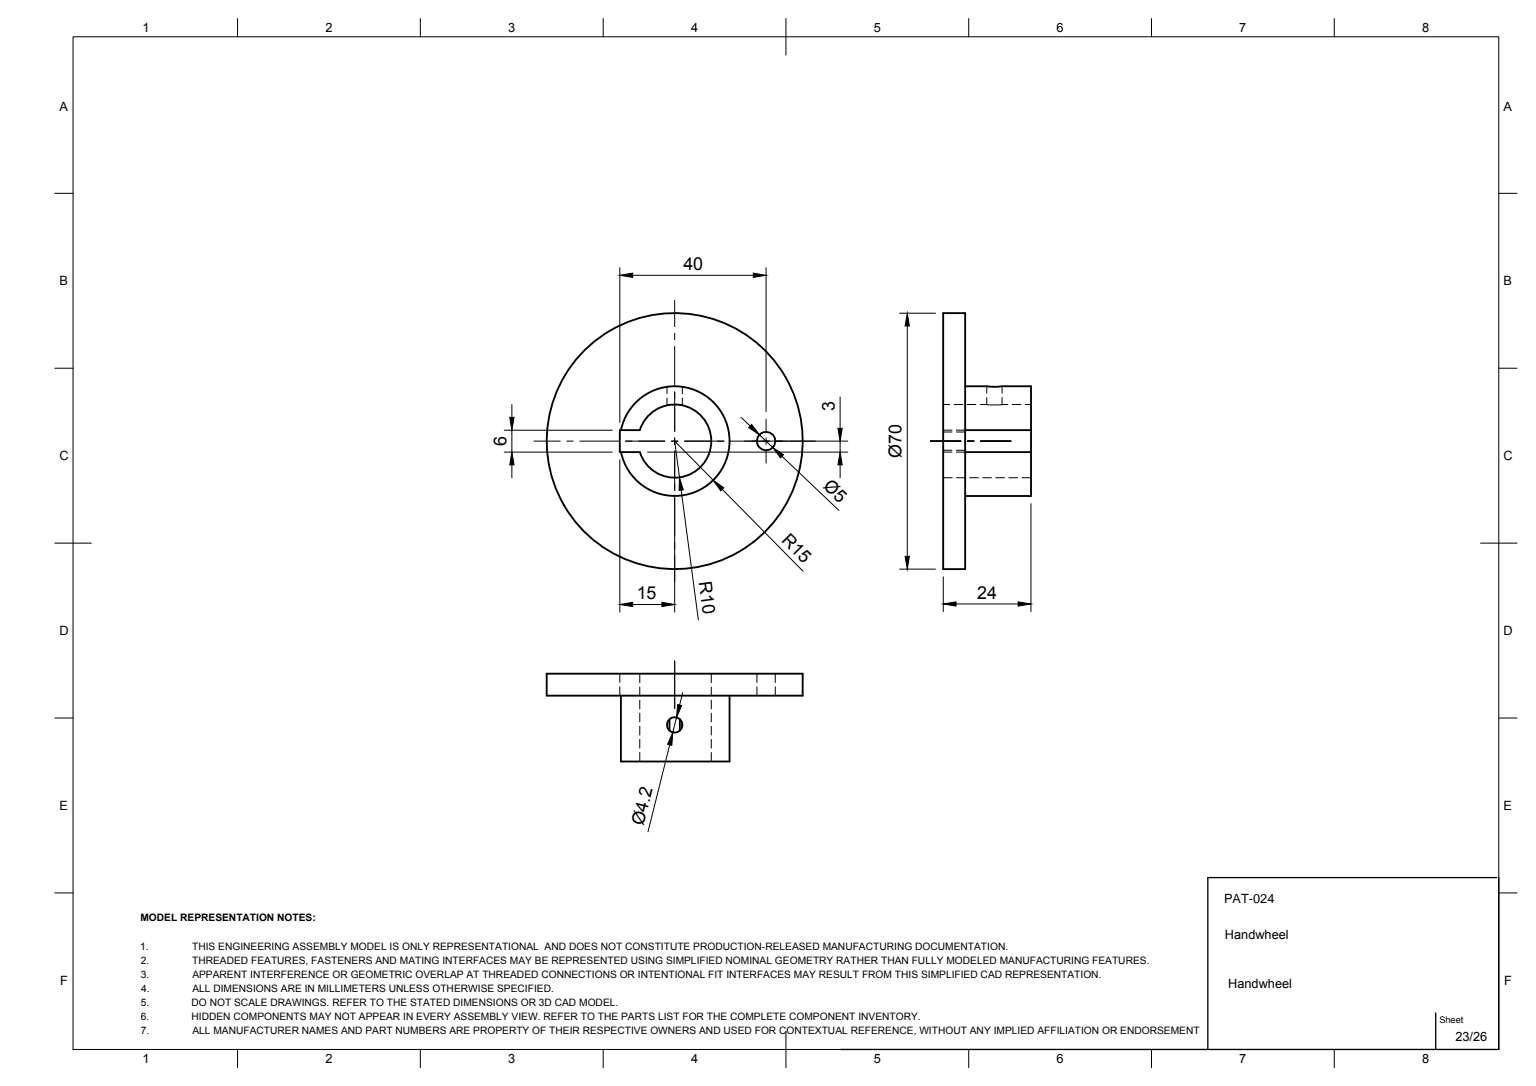
ISO-10303-21;
HEADER;
/* Generated by software containing ST-Developer
 * from STEP Tools, Inc. (www.steptools.com) 
 */

FILE_DESCRIPTION(
/* description */ ('Compact handwheel screw vise'),
/* implementation_level */ '2;1');

FILE_NAME(
/* name */ 'Handwheel.step',
/* time_stamp */ '2026-10-29T16:08:22-07:00',
/* author */ (''),
/* organization */ (''),
/* preprocessor_version */ 'ST-DEVELOPER v20.2',
/* originating_system */ 'Autodesk Translation Framework v15.17.0.0',
/* authorisation */ '');

FILE_SCHEMA (('AUTOMOTIVE_DESIGN { 1 0 10303 214 3 1 1 }'));
ENDSEC;

DATA;
#10=MECHANICAL_DESIGN_GEOMETRIC_PRESENTATION_REPRESENTATION('',(#673),#25074);
#536=B_SPLINE_CURVE_WITH_KNOTS('',3,(#24645,#24646,#24647,#24648,#24649,
#24650),.UNSPECIFIED.,.F.,.F.,(4,2,4),(0.803821788694078,0.872950991853625,
0.952307212900975),.UNSPECIFIED.);
#537=B_SPLINE_CURVE_WITH_KNOTS('',3,(#24653,#24654,#24655,#24656,#24657,
#24658,#24659,#24660,#24661,#24662),.UNSPECIFIED.,.F.,.F.,(4,2,2,2,4),(0.168950313426762,
0.238079516586309,0.317435737633658,0.396791958681008,0.465921161840561),
 .UNSPECIFIED.);
#538=B_SPLINE_CURVE_WITH_KNOTS('',3,(#24663,#24664,#24665,#24666,#24667,
#24668),.UNSPECIFIED.,.F.,.F.,(4,2,4),(0.952307212900975,1.03166343394832,
1.10079263710787),.UNSPECIFIED.);
#539=B_SPLINE_CURVE_WITH_KNOTS('',3,(#24672,#24673,#24674,#24675,#24676,
#24677,#24678,#24679,#24680,#24681),.UNSPECIFIED.,.F.,.F.,(4,2,2,2,4),(0.,
0.0792165807733642,0.158433161546728,0.237648697074572,0.316864232602417),
 .UNSPECIFIED.);
#540=B_SPLINE_CURVE_WITH_KNOTS('',3,(#24682,#24683,#24684,#24685,#24686,
#24687,#24688,#24689,#24690,#24691,#24692,#24693,#24694,#24695,#24696,#24697,
#24698,#24699,#24700,#24701,#24702,#24703,#24704,#24705,#24706,#24707),
 .UNSPECIFIED.,.F.,.F.,(4,2,2,2,2,2,2,2,2,2,2,2,4),(0.316864232602417,0.396079768130261,
0.475295303658105,0.554511884431469,0.633728465204833,0.712945045978197,
0.792161626751562,0.871377162279406,0.95059269780725,1.02980823333509,1.10902376886294,
1.1882403496363,1.26745693040967),.UNSPECIFIED.);
#609=SHAPE_REPRESENTATION_RELATIONSHIP('SRR','None',#25220,#637);
#637=ADVANCED_BREP_SHAPE_REPRESENTATION('',(#706),#25067);
#673=STYLED_ITEM('',(#25432),#706);
#706=MANIFOLD_SOLID_BREP('Body1',#8084);
#808=FACE_BOUND('',#1992,.T.);
#809=FACE_BOUND('',#1993,.T.);
#810=FACE_BOUND('',#1995,.T.);
#811=FACE_BOUND('',#1996,.T.);
#812=FACE_BOUND('',#1999,.T.);
#813=FACE_BOUND('',#2001,.T.);
#968=PLANE('',#9070);
#969=PLANE('',#9074);
#970=PLANE('',#9075);
#971=PLANE('',#9076);
#972=PLANE('',#9077);
#973=PLANE('',#9078);
#974=PLANE('',#9081);
#975=PLANE('',#9089);
#1418=FACE_OUTER_BOUND('',#1984,.T.);
#1419=FACE_OUTER_BOUND('',#1985,.T.);
#1420=FACE_OUTER_BOUND('',#1986,.T.);
#1421=FACE_OUTER_BOUND('',#1987,.T.);
#1422=FACE_OUTER_BOUND('',#1988,.T.);
#1423=FACE_OUTER_BOUND('',#1989,.T.);
#1424=FACE_OUTER_BOUND('',#1990,.T.);
#1425=FACE_OUTER_BOUND('',#1991,.T.);
#1426=FACE_OUTER_BOUND('',#1994,.T.);
#1427=FACE_OUTER_BOUND('',#1997,.T.);
#1428=FACE_OUTER_BOUND('',#1998,.T.);
#1429=FACE_OUTER_BOUND('',#2000,.T.);
#1430=FACE_OUTER_BOUND('',#2002,.T.);
#1984=EDGE_LOOP('',(#7079,#7080,#7081,#7082));
#1985=EDGE_LOOP('',(#7083,#7084));
#1986=EDGE_LOOP('',(#7085,#7086,#7087,#7088,#7089,#7090,#7091,#7092,#7093));
#1987=EDGE_LOOP('',(#7094,#7095));
#1988=EDGE_LOOP('',(#7096,#7097,#7098,#7099,#7100,#7101));
#1989=EDGE_LOOP('',(#7102,#7103,#7104,#7105));
#1990=EDGE_LOOP('',(#7106,#7107,#7108,#7109,#7110,#7111));
#1991=EDGE_LOOP('',(#7112));
#1992=EDGE_LOOP('',(#7113));
#1993=EDGE_LOOP('',(#7114,#7115,#7116,#7117));
#1994=EDGE_LOOP('',(#7118));
#1995=EDGE_LOOP('',(#7119));
#1996=EDGE_LOOP('',(#7120,#7121,#7122,#7123));
#1997=EDGE_LOOP('',(#7124,#7125,#7126,#7127));
#1998=EDGE_LOOP('',(#7128,#7129,#7130,#7131));
#1999=EDGE_LOOP('',(#7132,#7133,#7134,#7135,#7136));
#2000=EDGE_LOOP('',(#7137,#7138,#7139,#7140));
#2001=EDGE_LOOP('',(#7141,#7142));
#2002=EDGE_LOOP('',(#7143,#7144,#7145,#7146));
#2476=LINE('',#24635,#2984);
#2477=LINE('',#24640,#2985);
#2478=LINE('',#24670,#2986);
#2479=LINE('',#24709,#2987);
#2480=LINE('',#24713,#2988);
#2481=LINE('',#24715,#2989);
#2482=LINE('',#24717,#2990);
#2483=LINE('',#24719,#2991);
#2484=LINE('',#24721,#2992);
#2485=LINE('',#24722,#2993);
#2486=LINE('',#24725,#2994);
#2487=LINE('',#24727,#2995);
#2488=LINE('',#24728,#2996);
#2489=LINE('',#24731,#2997);
#2490=LINE('',#24733,#2998);
#2491=LINE('',#24735,#2999);
#2492=LINE('',#24737,#3000);
#2493=LINE('',#24738,#3001);
#2494=LINE('',#24748,#3002);
#2984=VECTOR('',#10954,0.25);
#2985=VECTOR('',#10959,1.);
#2986=VECTOR('',#10966,0.210000000000001);
#2987=VECTOR('',#10969,1.);
#2988=VECTOR('',#10972,1.);
#2989=VECTOR('',#10973,1.);
#2990=VECTOR('',#10974,1.);
#2991=VECTOR('',#10975,1.);
#2992=VECTOR('',#10976,1.);
#2993=VECTOR('',#10977,1.);
#2994=VECTOR('',#10980,1.);
#2995=VECTOR('',#10981,1.);
#2996=VECTOR('',#10982,1.);
#2997=VECTOR('',#10985,1.);
#2998=VECTOR('',#10986,1.);
#2999=VECTOR('',#10987,1.);
#3000=VECTOR('',#10988,1.);
#3001=VECTOR('',#10989,1.);
#3002=VECTOR('',#11004,3.5);
#3299=CIRCLE('',#9068,0.25);
#3300=CIRCLE('',#9069,0.25);
#3301=CIRCLE('',#9071,0.210000000000001);
#3302=CIRCLE('',#9073,0.210000000000001);
#3303=CIRCLE('',#9079,3.5);
#3304=CIRCLE('',#9080,1.);
#3305=CIRCLE('',#9082,3.5);
#3306=CIRCLE('',#9083,1.5);
#3307=CIRCLE('',#9086,1.);
#3308=CIRCLE('',#9088,1.5);
#3979=VERTEX_POINT('',#24632);
#3980=VERTEX_POINT('',#24634);
#3981=VERTEX_POINT('',#24638);
#3982=VERTEX_POINT('',#24639);
#3983=VERTEX_POINT('',#24643);
#3984=VERTEX_POINT('',#24644);
#3985=VERTEX_POINT('',#24651);
#3986=VERTEX_POINT('',#24669);
#3987=VERTEX_POINT('',#24671);
#3988=VERTEX_POINT('',#24711);
#3989=VERTEX_POINT('',#24712);
#3990=VERTEX_POINT('',#24714);
#3991=VERTEX_POINT('',#24716);
#3992=VERTEX_POINT('',#24718);
#3993=VERTEX_POINT('',#24720);
#3994=VERTEX_POINT('',#24724);
#3995=VERTEX_POINT('',#24726);
#3996=VERTEX_POINT('',#24730);
#3997=VERTEX_POINT('',#24732);
#3998=VERTEX_POINT('',#24734);
#3999=VERTEX_POINT('',#24736);
#4000=VERTEX_POINT('',#24740);
#4001=VERTEX_POINT('',#24744);
#5026=EDGE_CURVE('',#3979,#3979,#3299,.T.);
#5027=EDGE_CURVE('',#3979,#3980,#2476,.T.);
#5028=EDGE_CURVE('',#3980,#3980,#3300,.T.);
#5029=EDGE_CURVE('',#3981,#3982,#2477,.T.);
#5030=EDGE_CURVE('',#3981,#3982,#3301,.T.);
#5031=EDGE_CURVE('',#3983,#3984,#536,.T.);
#5032=EDGE_CURVE('',#3985,#3983,#3302,.T.);
#5033=EDGE_CURVE('',#3982,#3985,#537,.T.);
#5034=EDGE_CURVE('',#3984,#3981,#538,.T.);
#5035=EDGE_CURVE('',#3984,#3986,#2478,.T.);
#5036=EDGE_CURVE('',#3987,#3986,#539,.T.);
#5037=EDGE_CURVE('',#3986,#3987,#540,.T.);
#5038=EDGE_CURVE('',#3985,#3983,#2479,.T.);
#5039=EDGE_CURVE('',#3988,#3989,#2480,.T.);
#5040=EDGE_CURVE('',#3990,#3988,#2481,.T.);
#5041=EDGE_CURVE('',#3991,#3990,#2482,.T.);
#5042=EDGE_CURVE('',#3992,#3991,#2483,.T.);
#5043=EDGE_CURVE('',#3993,#3992,#2484,.T.);
#5044=EDGE_CURVE('',#3989,#3993,#2485,.T.);
#5045=EDGE_CURVE('',#3994,#3988,#2486,.T.);
#5046=EDGE_CURVE('',#3995,#3994,#2487,.T.);
#5047=EDGE_CURVE('',#3990,#3995,#2488,.T.);
#5048=EDGE_CURVE('',#3996,#3994,#2489,.T.);
#5049=EDGE_CURVE('',#3997,#3996,#2490,.T.);
#5050=EDGE_CURVE('',#3998,#3997,#2491,.T.);
#5051=EDGE_CURVE('',#3999,#3998,#2492,.T.);
#5052=EDGE_CURVE('',#3995,#3999,#2493,.T.);
#5053=EDGE_CURVE('',#4000,#4000,#3303,.T.);
#5054=EDGE_CURVE('',#3989,#3996,#3304,.T.);
#5055=EDGE_CURVE('',#4001,#4001,#3305,.T.);
#5056=EDGE_CURVE('',#3999,#3991,#3306,.T.);
#5057=EDGE_CURVE('',#4000,#4001,#2494,.T.);
#5058=EDGE_CURVE('',#3993,#3997,#3307,.T.);
#5059=EDGE_CURVE('',#3998,#3992,#3308,.T.);
#7079=ORIENTED_EDGE('',*,*,#5026,.F.);
#7080=ORIENTED_EDGE('',*,*,#5027,.T.);
#7081=ORIENTED_EDGE('',*,*,#5028,.F.);
#7082=ORIENTED_EDGE('',*,*,#5027,.F.);
#7083=ORIENTED_EDGE('',*,*,#5029,.F.);
#7084=ORIENTED_EDGE('',*,*,#5030,.T.);
#7085=ORIENTED_EDGE('',*,*,#5031,.F.);
#7086=ORIENTED_EDGE('',*,*,#5032,.F.);
#7087=ORIENTED_EDGE('',*,*,#5033,.F.);
#7088=ORIENTED_EDGE('',*,*,#5030,.F.);
#7089=ORIENTED_EDGE('',*,*,#5034,.F.);
#7090=ORIENTED_EDGE('',*,*,#5035,.T.);
#7091=ORIENTED_EDGE('',*,*,#5036,.F.);
#7092=ORIENTED_EDGE('',*,*,#5037,.F.);
#7093=ORIENTED_EDGE('',*,*,#5035,.F.);
#7094=ORIENTED_EDGE('',*,*,#5038,.F.);
#7095=ORIENTED_EDGE('',*,*,#5032,.T.);
#7096=ORIENTED_EDGE('',*,*,#5039,.F.);
#7097=ORIENTED_EDGE('',*,*,#5040,.F.);
#7098=ORIENTED_EDGE('',*,*,#5041,.F.);
#7099=ORIENTED_EDGE('',*,*,#5042,.F.);
#7100=ORIENTED_EDGE('',*,*,#5043,.F.);
#7101=ORIENTED_EDGE('',*,*,#5044,.F.);
#7102=ORIENTED_EDGE('',*,*,#5045,.F.);
#7103=ORIENTED_EDGE('',*,*,#5046,.F.);
#7104=ORIENTED_EDGE('',*,*,#5047,.F.);
#7105=ORIENTED_EDGE('',*,*,#5040,.T.);
#7106=ORIENTED_EDGE('',*,*,#5048,.F.);
#7107=ORIENTED_EDGE('',*,*,#5049,.F.);
#7108=ORIENTED_EDGE('',*,*,#5050,.F.);
#7109=ORIENTED_EDGE('',*,*,#5051,.F.);
#7110=ORIENTED_EDGE('',*,*,#5052,.F.);
#7111=ORIENTED_EDGE('',*,*,#5046,.T.);
#7112=ORIENTED_EDGE('',*,*,#5053,.T.);
#7113=ORIENTED_EDGE('',*,*,#5028,.T.);
#7114=ORIENTED_EDGE('',*,*,#5048,.T.);
#7115=ORIENTED_EDGE('',*,*,#5045,.T.);
#7116=ORIENTED_EDGE('',*,*,#5039,.T.);
#7117=ORIENTED_EDGE('',*,*,#5054,.T.);
#7118=ORIENTED_EDGE('',*,*,#5055,.F.);
#7119=ORIENTED_EDGE('',*,*,#5026,.T.);
#7120=ORIENTED_EDGE('',*,*,#5052,.T.);
#7121=ORIENTED_EDGE('',*,*,#5056,.T.);
#7122=ORIENTED_EDGE('',*,*,#5041,.T.);
#7123=ORIENTED_EDGE('',*,*,#5047,.T.);
#7124=ORIENTED_EDGE('',*,*,#5053,.F.);
#7125=ORIENTED_EDGE('',*,*,#5057,.T.);
#7126=ORIENTED_EDGE('',*,*,#5055,.T.);
#7127=ORIENTED_EDGE('',*,*,#5057,.F.);
#7128=ORIENTED_EDGE('',*,*,#5049,.T.);
#7129=ORIENTED_EDGE('',*,*,#5054,.F.);
#7130=ORIENTED_EDGE('',*,*,#5044,.T.);
#7131=ORIENTED_EDGE('',*,*,#5058,.T.);
#7132=ORIENTED_EDGE('',*,*,#5033,.T.);
#7133=ORIENTED_EDGE('',*,*,#5038,.T.);
#7134=ORIENTED_EDGE('',*,*,#5031,.T.);
#7135=ORIENTED_EDGE('',*,*,#5034,.T.);
#7136=ORIENTED_EDGE('',*,*,#5029,.T.);
#7137=ORIENTED_EDGE('',*,*,#5051,.T.);
#7138=ORIENTED_EDGE('',*,*,#5059,.T.);
#7139=ORIENTED_EDGE('',*,*,#5042,.T.);
#7140=ORIENTED_EDGE('',*,*,#5056,.F.);
#7141=ORIENTED_EDGE('',*,*,#5036,.T.);
#7142=ORIENTED_EDGE('',*,*,#5037,.T.);
#7143=ORIENTED_EDGE('',*,*,#5050,.T.);
#7144=ORIENTED_EDGE('',*,*,#5058,.F.);
#7145=ORIENTED_EDGE('',*,*,#5043,.T.);
#7146=ORIENTED_EDGE('',*,*,#5059,.F.);
#7568=CYLINDRICAL_SURFACE('',#9067,0.25);
#7569=CYLINDRICAL_SURFACE('',#9072,0.210000000000001);
#7570=CYLINDRICAL_SURFACE('',#9084,3.5);
#7571=CYLINDRICAL_SURFACE('',#9085,1.);
#7572=CYLINDRICAL_SURFACE('',#9087,1.5);
#7988=ADVANCED_FACE('',(#1418),#7568,.F.);
#7989=ADVANCED_FACE('',(#1419),#968,.T.);
#7990=ADVANCED_FACE('',(#1420),#7569,.F.);
#7991=ADVANCED_FACE('',(#1421),#969,.T.);
#7992=ADVANCED_FACE('',(#1422),#970,.F.);
#7993=ADVANCED_FACE('',(#1423),#971,.F.);
#7994=ADVANCED_FACE('',(#1424),#972,.F.);
#7995=ADVANCED_FACE('',(#1425,#808,#809),#973,.T.);
#7996=ADVANCED_FACE('',(#1426,#810,#811),#974,.F.);
#7997=ADVANCED_FACE('',(#1427),#7570,.T.);
#7998=ADVANCED_FACE('',(#1428,#812),#7571,.F.);
#7999=ADVANCED_FACE('',(#1429,#813),#7572,.T.);
#8000=ADVANCED_FACE('',(#1430),#975,.F.);
#8084=CLOSED_SHELL('',(#7988,#7989,#7990,#7991,#7992,#7993,#7994,#7995,
#7996,#7997,#7998,#7999,#8000));
#9066=AXIS2_PLACEMENT_3D('',#24630,#10948,#10949);
#9067=AXIS2_PLACEMENT_3D('',#24631,#10950,#10951);
#9068=AXIS2_PLACEMENT_3D('',#24633,#10952,#10953);
#9069=AXIS2_PLACEMENT_3D('',#24636,#10955,#10956);
#9070=AXIS2_PLACEMENT_3D('',#24637,#10957,#10958);
#9071=AXIS2_PLACEMENT_3D('',#24641,#10960,#10961);
#9072=AXIS2_PLACEMENT_3D('',#24642,#10962,#10963);
#9073=AXIS2_PLACEMENT_3D('',#24652,#10964,#10965);
#9074=AXIS2_PLACEMENT_3D('',#24708,#10967,#10968);
#9075=AXIS2_PLACEMENT_3D('',#24710,#10970,#10971);
#9076=AXIS2_PLACEMENT_3D('',#24723,#10978,#10979);
#9077=AXIS2_PLACEMENT_3D('',#24729,#10983,#10984);
#9078=AXIS2_PLACEMENT_3D('',#24739,#10990,#10991);
#9079=AXIS2_PLACEMENT_3D('',#24741,#10992,#10993);
#9080=AXIS2_PLACEMENT_3D('',#24742,#10994,#10995);
#9081=AXIS2_PLACEMENT_3D('',#24743,#10996,#10997);
#9082=AXIS2_PLACEMENT_3D('',#24745,#10998,#10999);
#9083=AXIS2_PLACEMENT_3D('',#24746,#11000,#11001);
#9084=AXIS2_PLACEMENT_3D('',#24747,#11002,#11003);
#9085=AXIS2_PLACEMENT_3D('',#24749,#11005,#11006);
#9086=AXIS2_PLACEMENT_3D('',#24750,#11007,#11008);
#9087=AXIS2_PLACEMENT_3D('',#24751,#11009,#11010);
#9088=AXIS2_PLACEMENT_3D('',#24752,#11011,#11012);
#9089=AXIS2_PLACEMENT_3D('',#24753,#11013,#11014);
#10948=DIRECTION('axis',(0.,0.,1.));
#10949=DIRECTION('refdir',(1.,0.,0.));
#10950=DIRECTION('center_axis',(1.,0.,0.));
#10951=DIRECTION('ref_axis',(0.,0.,-1.));
#10952=DIRECTION('center_axis',(1.,0.,0.));
#10953=DIRECTION('ref_axis',(0.,0.,-1.));
#10954=DIRECTION('',(1.,0.,0.));
#10955=DIRECTION('center_axis',(-1.,0.,0.));
#10956=DIRECTION('ref_axis',(0.,0.,-1.));
#10957=DIRECTION('center_axis',(0.,1.,0.));
#10958=DIRECTION('ref_axis',(1.,0.,0.));
#10959=DIRECTION('',(1.,0.,0.));
#10960=DIRECTION('center_axis',(0.,1.,0.));
#10961=DIRECTION('ref_axis',(1.,0.,0.));
#10962=DIRECTION('center_axis',(0.,1.,0.));
#10963=DIRECTION('ref_axis',(1.,0.,0.));
#10964=DIRECTION('center_axis',(0.,1.,0.));
#10965=DIRECTION('ref_axis',(1.,0.,0.));
#10966=DIRECTION('',(0.,1.,0.));
#10967=DIRECTION('center_axis',(0.,1.,0.));
#10968=DIRECTION('ref_axis',(1.,0.,0.));
#10969=DIRECTION('',(-1.,0.,0.));
#10970=DIRECTION('center_axis',(0.,-1.,0.));
#10971=DIRECTION('ref_axis',(0.,0.,-1.));
#10972=DIRECTION('',(0.,0.,1.));
#10973=DIRECTION('',(1.,0.,0.));
#10974=DIRECTION('',(0.,0.,-1.));
#10975=DIRECTION('',(1.,0.,0.));
#10976=DIRECTION('',(0.,0.,-1.));
#10977=DIRECTION('',(-1.,0.,0.));
#10978=DIRECTION('center_axis',(0.,0.,-1.));
#10979=DIRECTION('ref_axis',(0.,1.,0.));
#10980=DIRECTION('',(0.,-1.,0.));
#10981=DIRECTION('',(1.,0.,0.));
#10982=DIRECTION('',(0.,1.,0.));
#10983=DIRECTION('center_axis',(0.,1.,0.));
#10984=DIRECTION('ref_axis',(0.,0.,1.));
#10985=DIRECTION('',(0.,0.,-1.));
#10986=DIRECTION('',(1.,0.,0.));
#10987=DIRECTION('',(0.,0.,1.));
#10988=DIRECTION('',(-1.,0.,0.));
#10989=DIRECTION('',(0.,0.,1.));
#10990=DIRECTION('center_axis',(1.,0.,0.));
#10991=DIRECTION('ref_axis',(0.,0.,-1.));
#10992=DIRECTION('center_axis',(1.,0.,0.));
#10993=DIRECTION('ref_axis',(0.,0.,-1.));
#10994=DIRECTION('center_axis',(-1.,0.,0.));
#10995=DIRECTION('ref_axis',(0.,0.,-1.));
#10996=DIRECTION('center_axis',(1.,0.,0.));
#10997=DIRECTION('ref_axis',(0.,0.,-1.));
#10998=DIRECTION('center_axis',(1.,0.,0.));
#10999=DIRECTION('ref_axis',(0.,0.,-1.));
#11000=DIRECTION('center_axis',(1.,0.,0.));
#11001=DIRECTION('ref_axis',(0.,0.,-1.));
#11002=DIRECTION('center_axis',(1.,0.,0.));
#11003=DIRECTION('ref_axis',(0.,0.,-1.));
#11004=DIRECTION('',(-1.,0.,0.));
#11005=DIRECTION('center_axis',(1.,0.,0.));
#11006=DIRECTION('ref_axis',(0.,1.22464679914735E-16,1.));
#11007=DIRECTION('center_axis',(-1.,0.,0.));
#11008=DIRECTION('ref_axis',(0.,0.,-1.));
#11009=DIRECTION('center_axis',(1.,0.,0.));
#11010=DIRECTION('ref_axis',(0.,1.22464679914735E-16,1.));
#11011=DIRECTION('center_axis',(1.,0.,0.));
#11012=DIRECTION('ref_axis',(0.,0.,-1.));
#11013=DIRECTION('center_axis',(1.,0.,0.));
#11014=DIRECTION('ref_axis',(0.,0.,-1.));
#24630=CARTESIAN_POINT('',(0.,0.,0.));
#24631=CARTESIAN_POINT('Origin',(28.7,0.,6.5));
#24632=CARTESIAN_POINT('',(28.8,-3.06161699786838E-17,6.75));
#24633=CARTESIAN_POINT('Origin',(28.8,0.,6.5));
#24634=CARTESIAN_POINT('',(29.4,3.06161699786838E-17,6.75));
#24635=CARTESIAN_POINT('',(28.7,-3.06161699786838E-17,6.75));
#24636=CARTESIAN_POINT('Origin',(29.4,0.,6.5));
#24637=CARTESIAN_POINT('Origin',(28.,0.99,4.));
#24638=CARTESIAN_POINT('',(27.844436508139,0.99,4.14106735979666));
#24639=CARTESIAN_POINT('',(28.155563491861,0.99,4.14106735979666));
#24640=CARTESIAN_POINT('',(27.,0.99,4.14106735979666));
#24641=CARTESIAN_POINT('Origin',(28.,0.99,4.));
#24642=CARTESIAN_POINT('Origin',(28.,0.99,4.));
#24643=CARTESIAN_POINT('',(27.844436508139,0.99,3.85893264020334));
#24644=CARTESIAN_POINT('',(27.79,1.,4.));
#24645=CARTESIAN_POINT('Ctrl Pts',(27.844436508139,0.99,3.85893264020334));
#24646=CARTESIAN_POINT('Ctrl Pts',(27.8287948476368,0.992457849824465,3.87618164330178));
#24647=CARTESIAN_POINT('Ctrl Pts',(27.815375956669,0.994938193049464,3.8970013568903));
#24648=CARTESIAN_POINT('Ctrl Pts',(27.7953025362756,0.998844492372413,3.94538588560165));
#24649=CARTESIAN_POINT('Ctrl Pts',(27.79,1.,3.97354792631755));
#24650=CARTESIAN_POINT('Ctrl Pts',(27.79,1.,4.));
#24651=CARTESIAN_POINT('',(28.155563491861,0.99,3.85893264020334));
#24652=CARTESIAN_POINT('Origin',(28.,0.99,4.));
#24653=CARTESIAN_POINT('Ctrl Pts',(28.155563491861,0.99,4.14106735979666));
#24654=CARTESIAN_POINT('Ctrl Pts',(28.1712051523632,0.992457849824465,4.12381835669823));
#24655=CARTESIAN_POINT('Ctrl Pts',(28.184624043331,0.994938193049464,4.1029986431097));
#24656=CARTESIAN_POINT('Ctrl Pts',(28.2046974637244,0.998844492372413,4.05461411439835));
#24657=CARTESIAN_POINT('Ctrl Pts',(28.21,1.,4.02645207368245));
#24658=CARTESIAN_POINT('Ctrl Pts',(28.21,1.,3.97354792631755));
#24659=CARTESIAN_POINT('Ctrl Pts',(28.2046974637244,0.998844492372413,3.94538588560165));
#24660=CARTESIAN_POINT('Ctrl Pts',(28.184624043331,0.994938193049464,3.8970013568903));
#24661=CARTESIAN_POINT('Ctrl Pts',(28.1712051523632,0.992457849824465,3.87618164330178));
#24662=CARTESIAN_POINT('Ctrl Pts',(28.155563491861,0.99,3.85893264020334));
#24663=CARTESIAN_POINT('Ctrl Pts',(27.79,1.,4.));
#24664=CARTESIAN_POINT('Ctrl Pts',(27.79,1.,4.02645207368245));
#24665=CARTESIAN_POINT('Ctrl Pts',(27.7953025362756,0.998844492372413,4.05461411439835));
#24666=CARTESIAN_POINT('Ctrl Pts',(27.815375956669,0.994938193049464,4.1029986431097));
#24667=CARTESIAN_POINT('Ctrl Pts',(27.8287948476368,0.992457849824465,4.12381835669823));
#24668=CARTESIAN_POINT('Ctrl Pts',(27.844436508139,0.99,4.14106735979666));
#24669=CARTESIAN_POINT('',(27.79,1.5,4.));
#24670=CARTESIAN_POINT('',(27.79,0.99,4.));
#24671=CARTESIAN_POINT('',(28.,1.48522725533839,4.21));
#24672=CARTESIAN_POINT('Ctrl Pts',(28.,1.48522725533839,4.21));
#24673=CARTESIAN_POINT('Ctrl Pts',(27.9735944730755,1.48522725533839,4.21));
#24674=CARTESIAN_POINT('Ctrl Pts',(27.9454529259093,1.48600415954412,4.20471573726959));
#24675=CARTESIAN_POINT('Ctrl Pts',(27.8937237310949,1.48880073282317,4.18327376303633));
#24676=CARTESIAN_POINT('Ctrl Pts',(27.870133075872,1.49077897157582,4.16711792397039));
#24677=CARTESIAN_POINT('Ctrl Pts',(27.832882321789,1.49448481141327,4.12986716988737));
#24678=CARTESIAN_POINT('Ctrl Pts',(27.8167262899986,1.49645455657129,4.10627640830576));
#24679=CARTESIAN_POINT('Ctrl Pts',(27.7952841751738,1.49923165515646,4.0545468514059));
#24680=CARTESIAN_POINT('Ctrl Pts',(27.79,1.5,4.02640517850928));
#24681=CARTESIAN_POINT('Ctrl Pts',(27.79,1.5,4.));
#24682=CARTESIAN_POINT('Ctrl Pts',(27.79,1.5,4.));
#24683=CARTESIAN_POINT('Ctrl Pts',(27.79,1.5,3.97359482149072));
#24684=CARTESIAN_POINT('Ctrl Pts',(27.7952841751738,1.49923165515646,3.9454531485941));
#24685=CARTESIAN_POINT('Ctrl Pts',(27.8167262899986,1.49645455657129,3.89372359169424));
#24686=CARTESIAN_POINT('Ctrl Pts',(27.832882321789,1.49448481141327,3.87013283011263));
#24687=CARTESIAN_POINT('Ctrl Pts',(27.870133075872,1.49077897157582,3.83288207602961));
#24688=CARTESIAN_POINT('Ctrl Pts',(27.8937237310949,1.48880073282317,3.81672623696367));
#24689=CARTESIAN_POINT('Ctrl Pts',(27.9454529259093,1.48600415954412,3.7952842627304));
#24690=CARTESIAN_POINT('Ctrl Pts',(27.9735944730755,1.48522725533839,3.79));
#24691=CARTESIAN_POINT('Ctrl Pts',(28.0264055269245,1.48522725533839,3.79));
#24692=CARTESIAN_POINT('Ctrl Pts',(28.0545470740907,1.48600415954412,3.7952842627304));
#24693=CARTESIAN_POINT('Ctrl Pts',(28.1062762689051,1.48880073282317,3.81672623696367));
#24694=CARTESIAN_POINT('Ctrl Pts',(28.129866924128,1.49077897157582,3.83288207602961));
#24695=CARTESIAN_POINT('Ctrl Pts',(28.167117678211,1.49448481141327,3.87013283011263));
#24696=CARTESIAN_POINT('Ctrl Pts',(28.1832737100014,1.49645455657129,3.89372359169424));
#24697=CARTESIAN_POINT('Ctrl Pts',(28.2047158248262,1.49923165515646,3.9454531485941));
#24698=CARTESIAN_POINT('Ctrl Pts',(28.21,1.5,3.97359482149072));
#24699=CARTESIAN_POINT('Ctrl Pts',(28.21,1.5,4.02640517850928));
#24700=CARTESIAN_POINT('Ctrl Pts',(28.2047158248262,1.49923165515646,4.0545468514059));
#24701=CARTESIAN_POINT('Ctrl Pts',(28.1832737100014,1.49645455657129,4.10627640830576));
#24702=CARTESIAN_POINT('Ctrl Pts',(28.167117678211,1.49448481141327,4.12986716988737));
#24703=CARTESIAN_POINT('Ctrl Pts',(28.129866924128,1.49077897157582,4.16711792397039));
#24704=CARTESIAN_POINT('Ctrl Pts',(28.1062762689051,1.48880073282317,4.18327376303633));
#24705=CARTESIAN_POINT('Ctrl Pts',(28.0545470740907,1.48600415954412,4.2047157372696));
#24706=CARTESIAN_POINT('Ctrl Pts',(28.0264055269245,1.48522725533839,4.21));
#24707=CARTESIAN_POINT('Ctrl Pts',(28.,1.48522725533839,4.21));
#24708=CARTESIAN_POINT('Origin',(28.,0.99,4.));
#24709=CARTESIAN_POINT('',(27.,0.99,3.85893264020334));
#24710=CARTESIAN_POINT('Origin',(26.9,-0.3,4.));
#24711=CARTESIAN_POINT('',(29.4,-0.3,2.5));
#24712=CARTESIAN_POINT('',(29.4,-0.3,3.04606079858305));
#24713=CARTESIAN_POINT('',(29.4,-0.3,4.));
#24714=CARTESIAN_POINT('',(28.8,-0.3,2.5));
#24715=CARTESIAN_POINT('',(26.9,-0.3,2.5));
#24716=CARTESIAN_POINT('',(28.8,-0.3,2.53030615433009));
#24717=CARTESIAN_POINT('',(28.8,-0.3,4.));
#24718=CARTESIAN_POINT('',(27.,-0.3,2.53030615433009));
#24719=CARTESIAN_POINT('',(27.,-0.3,2.53030615433009));
#24720=CARTESIAN_POINT('',(27.,-0.3,3.04606079858305));
#24721=CARTESIAN_POINT('',(27.,-0.3,4.));
#24722=CARTESIAN_POINT('',(27.,-0.3,3.04606079858305));
#24723=CARTESIAN_POINT('Origin',(26.9,-0.3,2.5));
#24724=CARTESIAN_POINT('',(29.4,0.3,2.5));
#24725=CARTESIAN_POINT('',(29.4,-0.15,2.5));
#24726=CARTESIAN_POINT('',(28.8,0.3,2.5));
#24727=CARTESIAN_POINT('',(26.9,0.3,2.5));
#24728=CARTESIAN_POINT('',(28.8,-0.15,2.5));
#24729=CARTESIAN_POINT('Origin',(26.9,0.3,2.5));
#24730=CARTESIAN_POINT('',(29.4,0.3,3.04606079858305));
#24731=CARTESIAN_POINT('',(29.4,0.3,3.25));
#24732=CARTESIAN_POINT('',(27.,0.3,3.04606079858305));
#24733=CARTESIAN_POINT('',(27.,0.3,3.04606079858305));
#24734=CARTESIAN_POINT('',(27.,0.3,2.53030615433009));
#24735=CARTESIAN_POINT('',(27.,0.3,3.25));
#24736=CARTESIAN_POINT('',(28.8,0.3,2.53030615433009));
#24737=CARTESIAN_POINT('',(27.,0.3,2.53030615433009));
#24738=CARTESIAN_POINT('',(28.8,0.3,3.25));
#24739=CARTESIAN_POINT('Origin',(29.4,0.,4.));
#24740=CARTESIAN_POINT('',(29.4,-4.28626379701574E-16,7.5));
#24741=CARTESIAN_POINT('Origin',(29.4,0.,4.));
#24742=CARTESIAN_POINT('Origin',(29.4,0.,4.));
#24743=CARTESIAN_POINT('Origin',(28.8,0.,4.));
#24744=CARTESIAN_POINT('',(28.8,-4.28626379701574E-16,7.5));
#24745=CARTESIAN_POINT('Origin',(28.8,0.,4.));
#24746=CARTESIAN_POINT('Origin',(28.8,0.,4.));
#24747=CARTESIAN_POINT('Origin',(28.8,0.,4.));
#24748=CARTESIAN_POINT('',(28.8,-4.28626379701574E-16,7.5));
#24749=CARTESIAN_POINT('Origin',(27.,0.,4.));
#24750=CARTESIAN_POINT('Origin',(27.,0.,4.));
#24751=CARTESIAN_POINT('Origin',(27.,0.,4.));
#24752=CARTESIAN_POINT('Origin',(27.,0.,4.));
#24753=CARTESIAN_POINT('Origin',(27.,0.,4.));
#25033=UNCERTAINTY_MEASURE_WITH_UNIT(LENGTH_MEASURE(0.001),#25075,
'DISTANCE_ACCURACY_VALUE',
'Maximum model space distance between geometric entities at asserted c
onnectivities');
#25040=UNCERTAINTY_MEASURE_WITH_UNIT(LENGTH_MEASURE(0.001),#25075,
'DISTANCE_ACCURACY_VALUE',
'Maximum model space distance between geometric entities at asserted c
onnectivities');
#25067=(
GEOMETRIC_REPRESENTATION_CONTEXT(3)
GLOBAL_UNCERTAINTY_ASSIGNED_CONTEXT((#25033))
GLOBAL_UNIT_ASSIGNED_CONTEXT((#25075,#25077,#25078))
REPRESENTATION_CONTEXT('','3D')
);
#25074=(
GEOMETRIC_REPRESENTATION_CONTEXT(3)
GLOBAL_UNCERTAINTY_ASSIGNED_CONTEXT((#25040))
GLOBAL_UNIT_ASSIGNED_CONTEXT((#25075,#25077,#25078))
REPRESENTATION_CONTEXT('','3D')
);
#25075=(
LENGTH_UNIT()
NAMED_UNIT(*)
SI_UNIT(.CENTI.,.METRE.)
);
#25077=(
NAMED_UNIT(*)
PLANE_ANGLE_UNIT()
SI_UNIT($,.RADIAN.)
);
#25078=(
NAMED_UNIT(*)
SI_UNIT($,.STERADIAN.)
SOLID_ANGLE_UNIT()
);
#25105=SHAPE_DEFINITION_REPRESENTATION(#25154,#25220);
#25154=PRODUCT_DEFINITION_SHAPE('',$,#25254);
#25220=SHAPE_REPRESENTATION('',(#9066),#25067);
#25227=PRODUCT_DEFINITION_CONTEXT('part definition',#25328,'design');
#25254=PRODUCT_DEFINITION('Handwheel','Handwheel',#25287,#25227);
#25287=PRODUCT_DEFINITION_FORMATION('',$,#25356);
#25328=APPLICATION_CONTEXT(
'Core Data for Automotive Mechanical Design Process');
#25329=PRODUCT_CONTEXT('part definition',#25328,'mechanical');
#25356=PRODUCT('Handwheel','Handwheel','Handwheel',(#25329));
#25426=COLOUR_RGB('Sky Blue',0.24,0.69,0.87);
#25427=FILL_AREA_STYLE_COLOUR('',#25426);
#25428=FILL_AREA_STYLE('',(#25427));
#25429=SURFACE_STYLE_FILL_AREA(#25428);
#25430=SURFACE_SIDE_STYLE('',(#25429));
#25431=SURFACE_STYLE_USAGE(.BOTH.,#25430);
#25432=PRESENTATION_STYLE_ASSIGNMENT((#25431));
ENDSEC;
END-ISO-10303-21;
